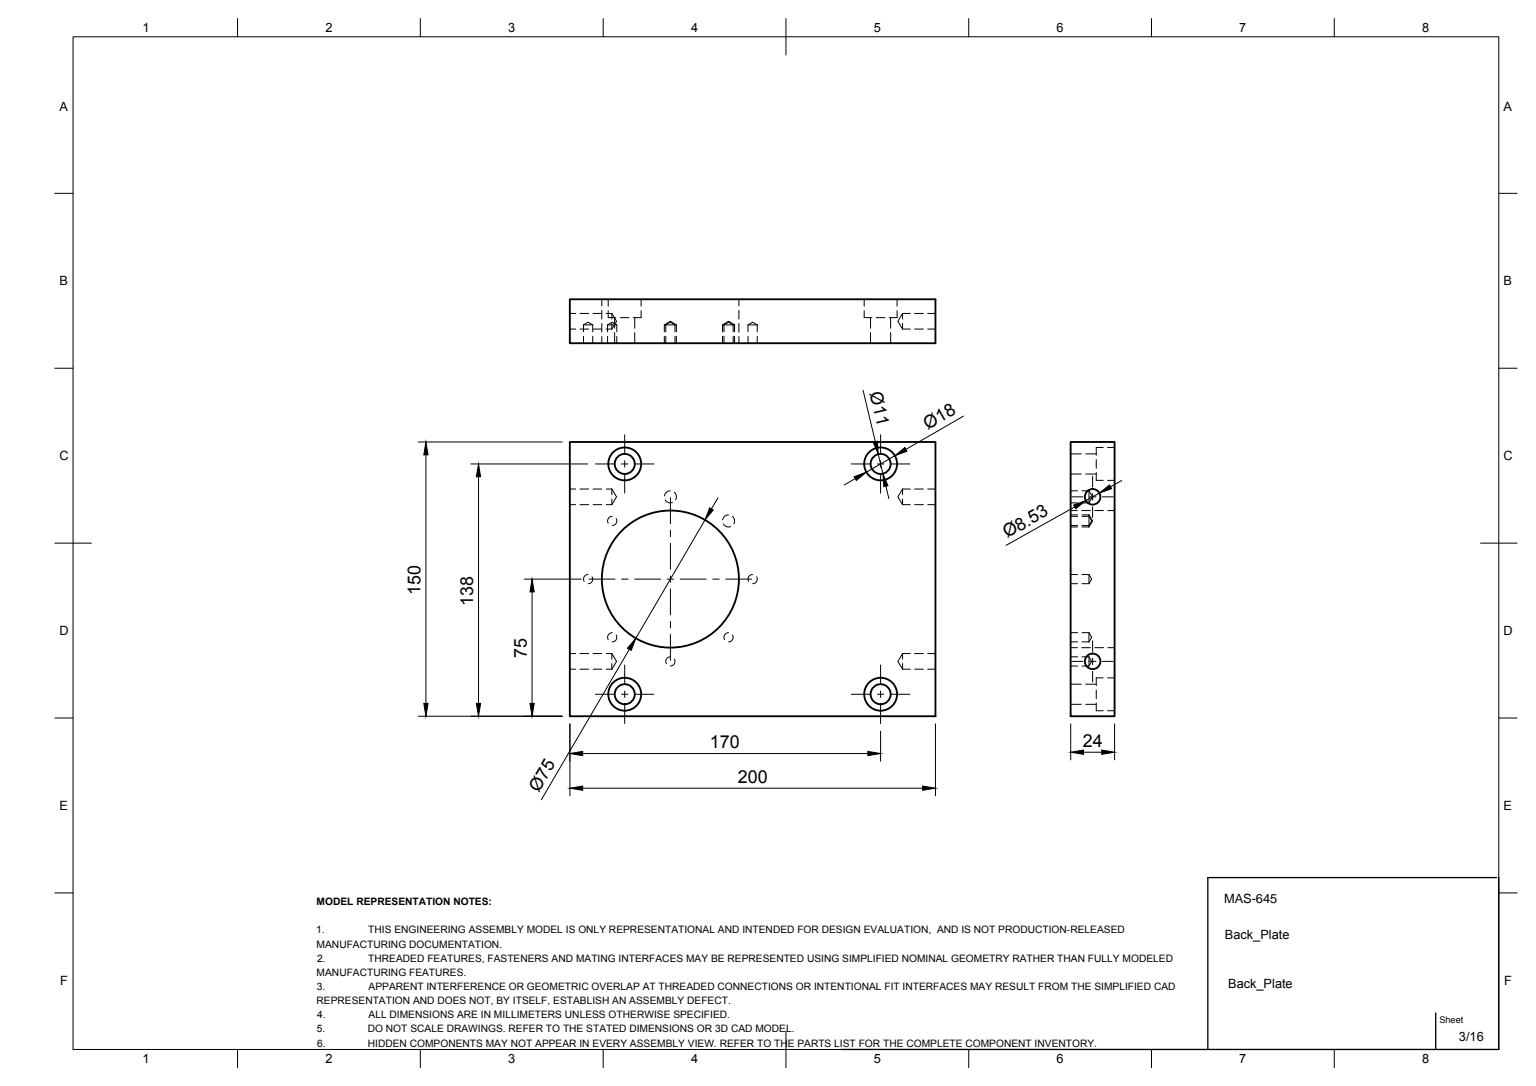
ISO-10303-21;
HEADER;
FILE_DESCRIPTION((''),'2;1');
FILE_NAME('Back_Plate.step','2026-10-09T10:54:55-07:00',(''),(''),'','','');
FILE_SCHEMA (('AUTOMOTIVE_DESIGN { 1 0 10303 214 3 1 1 }'));
ENDSEC;
DATA;
#10=MECHANICAL_DESIGN_GEOMETRIC_PRESENTATION_REPRESENTATION('',(#595),#63824);
#565=SHAPE_REPRESENTATION_RELATIONSHIP('SRR','None',#63879,#580) ;
#580=ADVANCED_BREP_SHAPE_REPRESENTATION('',(#610),#63809) ;
#595=STYLED_ITEM('',(#63963),#610) ;
#610=MANIFOLD_SOLID_BREP('Body1',#15494) ;
#625=FACE_BOUND('',#2415,.T.) ;
#626=FACE_BOUND('',#2419,.T.) ;
#627=FACE_BOUND('',#2423,.T.) ;
#628=FACE_BOUND('',#2427,.T.) ;
#629=FACE_BOUND('',#2448,.T.) ;
#630=FACE_BOUND('',#2449,.T.) ;
#631=FACE_BOUND('',#2452,.T.) ;
#632=FACE_BOUND('',#2453,.T.) ;
#633=FACE_BOUND('',#2456,.T.) ;
#634=FACE_BOUND('',#2457,.T.) ;
#635=FACE_BOUND('',#2458,.T.) ;
#636=FACE_BOUND('',#2459,.T.) ;
#637=FACE_BOUND('',#2460,.T.) ;
#638=FACE_BOUND('',#2462,.T.) ;
#639=FACE_BOUND('',#2463,.T.) ;
#640=FACE_BOUND('',#2464,.T.) ;
#641=FACE_BOUND('',#2465,.T.) ;
#642=FACE_BOUND('',#2466,.T.) ;
#643=FACE_BOUND('',#2467,.T.) ;
#644=FACE_BOUND('',#2468,.T.) ;
#645=FACE_BOUND('',#2469,.T.) ;
#646=FACE_BOUND('',#2470,.T.) ;
#647=FACE_BOUND('',#2471,.T.) ;
#648=FACE_BOUND('',#2472,.T.) ;
#649=FACE_BOUND('',#2473,.T.) ;
#650=FACE_BOUND('',#2474,.T.) ;
#832=PLANE('',#15693) ;
#833=PLANE('',#15700) ;
#834=PLANE('',#15707) ;
#835=PLANE('',#15714) ;
#836=PLANE('',#15756) ;
#837=PLANE('',#15757) ;
#838=PLANE('',#15758) ;
#839=PLANE('',#15759) ;
#840=PLANE('',#15760) ;
#841=PLANE('',#15761) ;
#1116=CYLINDRICAL_SURFACE('',#15679,4.263) ;
#1117=CYLINDRICAL_SURFACE('',#15683,4.263) ;
#1118=CYLINDRICAL_SURFACE('',#15687,4.263) ;
#1119=CYLINDRICAL_SURFACE('',#15691,4.263) ;
#1120=CYLINDRICAL_SURFACE('',#15696,9.) ;
#1121=CYLINDRICAL_SURFACE('',#15698,5.5) ;
#1122=CYLINDRICAL_SURFACE('',#15703,9.) ;
#1123=CYLINDRICAL_SURFACE('',#15705,5.5) ;
#1124=CYLINDRICAL_SURFACE('',#15710,9.) ;
#1125=CYLINDRICAL_SURFACE('',#15712,5.5) ;
#1126=CYLINDRICAL_SURFACE('',#15717,9.) ;
#1127=CYLINDRICAL_SURFACE('',#15719,5.5) ;
#1128=CYLINDRICAL_SURFACE('',#15723,3.3) ;
#1129=CYLINDRICAL_SURFACE('',#15727,2.5175) ;
#1130=CYLINDRICAL_SURFACE('',#15731,2.5175) ;
#1131=CYLINDRICAL_SURFACE('',#15735,2.5175) ;
#1132=CYLINDRICAL_SURFACE('',#15739,2.5175) ;
#1133=CYLINDRICAL_SURFACE('',#15743,2.5175) ;
#1134=CYLINDRICAL_SURFACE('',#15747,2.5175) ;
#1135=CYLINDRICAL_SURFACE('',#15751,3.3) ;
#1136=CYLINDRICAL_SURFACE('',#15753,37.5) ;
#1545=FACE_OUTER_BOUND('',#2406,.T.) ;
#1546=FACE_OUTER_BOUND('',#2407,.T.) ;
#1547=FACE_OUTER_BOUND('',#2408,.T.) ;
#1548=FACE_OUTER_BOUND('',#2409,.T.) ;
#1549=FACE_OUTER_BOUND('',#2410,.T.) ;
#1550=FACE_OUTER_BOUND('',#2411,.T.) ;
#1551=FACE_OUTER_BOUND('',#2412,.T.) ;
#1552=FACE_OUTER_BOUND('',#2413,.T.) ;
#1553=FACE_OUTER_BOUND('',#2414,.T.) ;
#1554=FACE_OUTER_BOUND('',#2416,.T.) ;
#1555=FACE_OUTER_BOUND('',#2417,.T.) ;
#1556=FACE_OUTER_BOUND('',#2418,.T.) ;
#1557=FACE_OUTER_BOUND('',#2420,.T.) ;
#1558=FACE_OUTER_BOUND('',#2421,.T.) ;
#1559=FACE_OUTER_BOUND('',#2422,.T.) ;
#1560=FACE_OUTER_BOUND('',#2424,.T.) ;
#1561=FACE_OUTER_BOUND('',#2425,.T.) ;
#1562=FACE_OUTER_BOUND('',#2426,.T.) ;
#1563=FACE_OUTER_BOUND('',#2428,.T.) ;
#1564=FACE_OUTER_BOUND('',#2429,.T.) ;
#1565=FACE_OUTER_BOUND('',#2430,.T.) ;
#1566=FACE_OUTER_BOUND('',#2431,.T.) ;
#1567=FACE_OUTER_BOUND('',#2432,.T.) ;
#1568=FACE_OUTER_BOUND('',#2433,.T.) ;
#1569=FACE_OUTER_BOUND('',#2434,.T.) ;
#1570=FACE_OUTER_BOUND('',#2435,.T.) ;
#1571=FACE_OUTER_BOUND('',#2436,.T.) ;
#1572=FACE_OUTER_BOUND('',#2437,.T.) ;
#1573=FACE_OUTER_BOUND('',#2438,.T.) ;
#1574=FACE_OUTER_BOUND('',#2439,.T.) ;
#1575=FACE_OUTER_BOUND('',#2440,.T.) ;
#1576=FACE_OUTER_BOUND('',#2441,.T.) ;
#1577=FACE_OUTER_BOUND('',#2442,.T.) ;
#1578=FACE_OUTER_BOUND('',#2443,.T.) ;
#1579=FACE_OUTER_BOUND('',#2444,.T.) ;
#1580=FACE_OUTER_BOUND('',#2445,.T.) ;
#1581=FACE_OUTER_BOUND('',#2446,.T.) ;
#1582=FACE_OUTER_BOUND('',#2447,.T.) ;
#1583=FACE_OUTER_BOUND('',#2450,.T.) ;
#1584=FACE_OUTER_BOUND('',#2451,.T.) ;
#1585=FACE_OUTER_BOUND('',#2454,.T.) ;
#1586=FACE_OUTER_BOUND('',#2455,.T.) ;
#1587=FACE_OUTER_BOUND('',#2461,.T.) ;
#2406=EDGE_LOOP('',(#9802,#9803,#9804)) ;
#2407=EDGE_LOOP('',(#9805,#9806,#9807,#9808)) ;
#2408=EDGE_LOOP('',(#9809,#9810,#9811)) ;
#2409=EDGE_LOOP('',(#9812,#9813,#9814,#9815)) ;
#2410=EDGE_LOOP('',(#9816,#9817,#9818)) ;
#2411=EDGE_LOOP('',(#9819,#9820,#9821,#9822)) ;
#2412=EDGE_LOOP('',(#9823,#9824,#9825)) ;
#2413=EDGE_LOOP('',(#9826,#9827,#9828,#9829)) ;
#2414=EDGE_LOOP('',(#9830)) ;
#2415=EDGE_LOOP('',(#9831)) ;
#2416=EDGE_LOOP('',(#9832,#9833,#9834,#9835)) ;
#2417=EDGE_LOOP('',(#9836,#9837,#9838,#9839)) ;
#2418=EDGE_LOOP('',(#9840)) ;
#2419=EDGE_LOOP('',(#9841)) ;
#2420=EDGE_LOOP('',(#9842,#9843,#9844,#9845)) ;
#2421=EDGE_LOOP('',(#9846,#9847,#9848,#9849)) ;
#2422=EDGE_LOOP('',(#9850)) ;
#2423=EDGE_LOOP('',(#9851)) ;
#2424=EDGE_LOOP('',(#9852,#9853,#9854,#9855)) ;
#2425=EDGE_LOOP('',(#9856,#9857,#9858,#9859)) ;
#2426=EDGE_LOOP('',(#9860)) ;
#2427=EDGE_LOOP('',(#9861)) ;
#2428=EDGE_LOOP('',(#9862,#9863,#9864,#9865)) ;
#2429=EDGE_LOOP('',(#9866,#9867,#9868,#9869)) ;
#2430=EDGE_LOOP('',(#9870,#9871,#9872)) ;
#2431=EDGE_LOOP('',(#9873,#9874,#9875,#9876)) ;
#2432=EDGE_LOOP('',(#9877,#9878,#9879)) ;
#2433=EDGE_LOOP('',(#9880,#9881,#9882,#9883)) ;
#2434=EDGE_LOOP('',(#9884,#9885,#9886)) ;
#2435=EDGE_LOOP('',(#9887,#9888,#9889,#9890)) ;
#2436=EDGE_LOOP('',(#9891,#9892,#9893)) ;
#2437=EDGE_LOOP('',(#9894,#9895,#9896,#9897)) ;
#2438=EDGE_LOOP('',(#9898,#9899,#9900)) ;
#2439=EDGE_LOOP('',(#9901,#9902,#9903,#9904)) ;
#2440=EDGE_LOOP('',(#9905,#9906,#9907)) ;
#2441=EDGE_LOOP('',(#9908,#9909,#9910,#9911)) ;
#2442=EDGE_LOOP('',(#9912,#9913,#9914)) ;
#2443=EDGE_LOOP('',(#9915,#9916,#9917,#9918)) ;
#2444=EDGE_LOOP('',(#9919,#9920,#9921)) ;
#2445=EDGE_LOOP('',(#9922,#9923,#9924,#9925)) ;
#2446=EDGE_LOOP('',(#9926,#9927,#9928,#9929)) ;
#2447=EDGE_LOOP('',(#9930,#9931,#9932,#9933)) ;
#2448=EDGE_LOOP('',(#9934)) ;
#2449=EDGE_LOOP('',(#9935)) ;
#2450=EDGE_LOOP('',(#9936,#9937,#9938,#9939)) ;
#2451=EDGE_LOOP('',(#9940,#9941,#9942,#9943)) ;
#2452=EDGE_LOOP('',(#9944)) ;
#2453=EDGE_LOOP('',(#9945)) ;
#2454=EDGE_LOOP('',(#9946,#9947,#9948,#9949)) ;
#2455=EDGE_LOOP('',(#9950,#9951,#9952,#9953)) ;
#2456=EDGE_LOOP('',(#9954)) ;
#2457=EDGE_LOOP('',(#9955)) ;
#2458=EDGE_LOOP('',(#9956)) ;
#2459=EDGE_LOOP('',(#9957)) ;
#2460=EDGE_LOOP('',(#9958)) ;
#2461=EDGE_LOOP('',(#9959,#9960,#9961,#9962)) ;
#2462=EDGE_LOOP('',(#9963)) ;
#2463=EDGE_LOOP('',(#9964)) ;
#2464=EDGE_LOOP('',(#9965)) ;
#2465=EDGE_LOOP('',(#9966)) ;
#2466=EDGE_LOOP('',(#9967)) ;
#2467=EDGE_LOOP('',(#9968)) ;
#2468=EDGE_LOOP('',(#9969)) ;
#2469=EDGE_LOOP('',(#9970)) ;
#2470=EDGE_LOOP('',(#9971)) ;
#2471=EDGE_LOOP('',(#9972)) ;
#2472=EDGE_LOOP('',(#9973)) ;
#2473=EDGE_LOOP('',(#9974)) ;
#2474=EDGE_LOOP('',(#9975)) ;
#3474=CIRCLE('',#15678,4.263) ;
#3475=CIRCLE('',#15680,4.263) ;
#3476=CIRCLE('',#15682,4.263) ;
#3477=CIRCLE('',#15684,4.263) ;
#3478=CIRCLE('',#15686,4.263) ;
#3479=CIRCLE('',#15688,4.263) ;
#3480=CIRCLE('',#15690,4.263) ;
#3481=CIRCLE('',#15692,4.263) ;
#3482=CIRCLE('',#15694,9.) ;
#3483=CIRCLE('',#15695,5.5) ;
#3484=CIRCLE('',#15697,9.) ;
#3485=CIRCLE('',#15699,5.5) ;
#3486=CIRCLE('',#15701,9.) ;
#3487=CIRCLE('',#15702,5.5) ;
#3488=CIRCLE('',#15704,9.) ;
#3489=CIRCLE('',#15706,5.5) ;
#3490=CIRCLE('',#15708,9.) ;
#3491=CIRCLE('',#15709,5.5) ;
#3492=CIRCLE('',#15711,9.) ;
#3493=CIRCLE('',#15713,5.5) ;
#3494=CIRCLE('',#15715,9.) ;
#3495=CIRCLE('',#15716,5.5) ;
#3496=CIRCLE('',#15718,9.) ;
#3497=CIRCLE('',#15720,5.5) ;
#3498=CIRCLE('',#15722,3.3) ;
#3499=CIRCLE('',#15724,3.3) ;
#3500=CIRCLE('',#15726,2.5175) ;
#3501=CIRCLE('',#15728,2.5175) ;
#3502=CIRCLE('',#15730,2.5175) ;
#3503=CIRCLE('',#15732,2.5175) ;
#3504=CIRCLE('',#15734,2.5175) ;
#3505=CIRCLE('',#15736,2.5175) ;
#3506=CIRCLE('',#15738,2.5175) ;
#3507=CIRCLE('',#15740,2.5175) ;
#3508=CIRCLE('',#15742,2.5175) ;
#3509=CIRCLE('',#15744,2.5175) ;
#3510=CIRCLE('',#15746,2.5175) ;
#3511=CIRCLE('',#15748,2.5175) ;
#3512=CIRCLE('',#15750,3.3) ;
#3513=CIRCLE('',#15752,3.3) ;
#3514=CIRCLE('',#15754,37.5) ;
#3515=CIRCLE('',#15755,37.5) ;
#4690=LINE('',#23017,#5346) ;
#4691=LINE('',#23022,#5347) ;
#4692=LINE('',#23026,#5348) ;
#4693=LINE('',#23031,#5349) ;
#4694=LINE('',#23035,#5350) ;
#4695=LINE('',#23040,#5351) ;
#4696=LINE('',#23044,#5352) ;
#4697=LINE('',#23049,#5353) ;
#4698=LINE('',#23058,#5354) ;
#4699=LINE('',#23061,#5355) ;
#4700=LINE('',#23071,#5356) ;
#4701=LINE('',#23074,#5357) ;
#4702=LINE('',#23084,#5358) ;
#4703=LINE('',#23087,#5359) ;
#4704=LINE('',#23097,#5360) ;
#4705=LINE('',#23100,#5361) ;
#4706=LINE('',#23105,#5362) ;
#4707=LINE('',#23110,#5363) ;
#4708=LINE('',#23114,#5364) ;
#4709=LINE('',#23119,#5365) ;
#4710=LINE('',#23123,#5366) ;
#4711=LINE('',#23128,#5367) ;
#4712=LINE('',#23132,#5368) ;
#4713=LINE('',#23137,#5369) ;
#4714=LINE('',#23141,#5370) ;
#4715=LINE('',#23146,#5371) ;
#4716=LINE('',#23150,#5372) ;
#4717=LINE('',#23155,#5373) ;
#4718=LINE('',#23159,#5374) ;
#4719=LINE('',#23164,#5375) ;
#4720=LINE('',#23168,#5376) ;
#4721=LINE('',#23173,#5377) ;
#4722=LINE('',#23178,#5378) ;
#4723=LINE('',#23183,#5379) ;
#4724=LINE('',#23185,#5380) ;
#4725=LINE('',#23187,#5381) ;
#4726=LINE('',#23188,#5382) ;
#4727=LINE('',#23191,#5383) ;
#4728=LINE('',#23193,#5384) ;
#4729=LINE('',#23194,#5385) ;
#4730=LINE('',#23197,#5386) ;
#4731=LINE('',#23199,#5387) ;
#4732=LINE('',#23200,#5388) ;
#4733=LINE('',#23202,#5389) ;
#4734=LINE('',#23203,#5390) ;
#5346=VECTOR('',#17908,2.42186816158307) ;
#5347=VECTOR('',#17915,4.263) ;
#5348=VECTOR('',#17918,2.42186816158307) ;
#5349=VECTOR('',#17925,4.263) ;
#5350=VECTOR('',#17928,2.42186816158307) ;
#5351=VECTOR('',#17935,4.263) ;
#5352=VECTOR('',#17938,2.42186816158307) ;
#5353=VECTOR('',#17945,4.263) ;
#5354=VECTOR('',#17956,9.) ;
#5355=VECTOR('',#17959,5.5) ;
#5356=VECTOR('',#17972,9.) ;
#5357=VECTOR('',#17975,5.5) ;
#5358=VECTOR('',#17988,9.) ;
#5359=VECTOR('',#17991,5.5) ;
#5360=VECTOR('',#18004,9.) ;
#5361=VECTOR('',#18007,5.5) ;
#5362=VECTOR('',#18012,1.65) ;
#5363=VECTOR('',#18019,3.3) ;
#5364=VECTOR('',#18022,1.44243074893998) ;
#5365=VECTOR('',#18029,2.5175) ;
#5366=VECTOR('',#18032,1.44243074893998) ;
#5367=VECTOR('',#18039,2.5175) ;
#5368=VECTOR('',#18042,1.44243074893998) ;
#5369=VECTOR('',#18049,2.5175) ;
#5370=VECTOR('',#18052,1.44243074893998) ;
#5371=VECTOR('',#18059,2.5175) ;
#5372=VECTOR('',#18062,1.44243074893998) ;
#5373=VECTOR('',#18069,2.5175) ;
#5374=VECTOR('',#18072,1.44243074893998) ;
#5375=VECTOR('',#18079,2.5175) ;
#5376=VECTOR('',#18082,1.65) ;
#5377=VECTOR('',#18089,3.3) ;
#5378=VECTOR('',#18094,37.5) ;
#5379=VECTOR('',#18099,10.) ;
#5380=VECTOR('',#18100,10.) ;
#5381=VECTOR('',#18101,10.) ;
#5382=VECTOR('',#18102,10.) ;
#5383=VECTOR('',#18105,10.) ;
#5384=VECTOR('',#18106,10.) ;
#5385=VECTOR('',#18107,10.) ;
#5386=VECTOR('',#18110,10.) ;
#5387=VECTOR('',#18111,10.) ;
#5388=VECTOR('',#18112,10.) ;
#5389=VECTOR('',#18115,10.) ;
#5390=VECTOR('',#18116,10.) ;
#6002=VERTEX_POINT('',#23015) ;
#6003=VERTEX_POINT('',#23016) ;
#6004=VERTEX_POINT('',#23020) ;
#6005=VERTEX_POINT('',#23024) ;
#6006=VERTEX_POINT('',#23025) ;
#6007=VERTEX_POINT('',#23029) ;
#6008=VERTEX_POINT('',#23033) ;
#6009=VERTEX_POINT('',#23034) ;
#6010=VERTEX_POINT('',#23038) ;
#6011=VERTEX_POINT('',#23042) ;
#6012=VERTEX_POINT('',#23043) ;
#6013=VERTEX_POINT('',#23047) ;
#6014=VERTEX_POINT('',#23051) ;
#6015=VERTEX_POINT('',#23053) ;
#6016=VERTEX_POINT('',#23056) ;
#6017=VERTEX_POINT('',#23060) ;
#6018=VERTEX_POINT('',#23064) ;
#6019=VERTEX_POINT('',#23066) ;
#6020=VERTEX_POINT('',#23069) ;
#6021=VERTEX_POINT('',#23073) ;
#6022=VERTEX_POINT('',#23077) ;
#6023=VERTEX_POINT('',#23079) ;
#6024=VERTEX_POINT('',#23082) ;
#6025=VERTEX_POINT('',#23086) ;
#6026=VERTEX_POINT('',#23090) ;
#6027=VERTEX_POINT('',#23092) ;
#6028=VERTEX_POINT('',#23095) ;
#6029=VERTEX_POINT('',#23099) ;
#6030=VERTEX_POINT('',#23103) ;
#6031=VERTEX_POINT('',#23104) ;
#6032=VERTEX_POINT('',#23108) ;
#6033=VERTEX_POINT('',#23112) ;
#6034=VERTEX_POINT('',#23113) ;
#6035=VERTEX_POINT('',#23117) ;
#6036=VERTEX_POINT('',#23121) ;
#6037=VERTEX_POINT('',#23122) ;
#6038=VERTEX_POINT('',#23126) ;
#6039=VERTEX_POINT('',#23130) ;
#6040=VERTEX_POINT('',#23131) ;
#6041=VERTEX_POINT('',#23135) ;
#6042=VERTEX_POINT('',#23139) ;
#6043=VERTEX_POINT('',#23140) ;
#6044=VERTEX_POINT('',#23144) ;
#6045=VERTEX_POINT('',#23148) ;
#6046=VERTEX_POINT('',#23149) ;
#6047=VERTEX_POINT('',#23153) ;
#6048=VERTEX_POINT('',#23157) ;
#6049=VERTEX_POINT('',#23158) ;
#6050=VERTEX_POINT('',#23162) ;
#6051=VERTEX_POINT('',#23166) ;
#6052=VERTEX_POINT('',#23167) ;
#6053=VERTEX_POINT('',#23171) ;
#6054=VERTEX_POINT('',#23175) ;
#6055=VERTEX_POINT('',#23177) ;
#6056=VERTEX_POINT('',#23181) ;
#6057=VERTEX_POINT('',#23182) ;
#6058=VERTEX_POINT('',#23184) ;
#6059=VERTEX_POINT('',#23186) ;
#6060=VERTEX_POINT('',#23190) ;
#6061=VERTEX_POINT('',#23192) ;
#6062=VERTEX_POINT('',#23196) ;
#6063=VERTEX_POINT('',#23198) ;
#7455=EDGE_CURVE('',#6002,#6003,#4690,.T.) ;
#7456=EDGE_CURVE('',#6003,#6003,#3474,.T.) ;
#7457=EDGE_CURVE('',#6004,#6004,#3475,.T.) ;
#7458=EDGE_CURVE('',#6004,#6003,#4691,.T.) ;
#7459=EDGE_CURVE('',#6005,#6006,#4692,.T.) ;
#7460=EDGE_CURVE('',#6006,#6006,#3476,.T.) ;
#7461=EDGE_CURVE('',#6007,#6007,#3477,.T.) ;
#7462=EDGE_CURVE('',#6007,#6006,#4693,.T.) ;
#7463=EDGE_CURVE('',#6008,#6009,#4694,.T.) ;
#7464=EDGE_CURVE('',#6009,#6009,#3478,.T.) ;
#7465=EDGE_CURVE('',#6010,#6010,#3479,.T.) ;
#7466=EDGE_CURVE('',#6010,#6009,#4695,.T.) ;
#7467=EDGE_CURVE('',#6011,#6012,#4696,.T.) ;
#7468=EDGE_CURVE('',#6012,#6012,#3480,.T.) ;
#7469=EDGE_CURVE('',#6013,#6013,#3481,.T.) ;
#7470=EDGE_CURVE('',#6013,#6012,#4697,.T.) ;
#7471=EDGE_CURVE('',#6014,#6014,#3482,.T.) ;
#7472=EDGE_CURVE('',#6015,#6015,#3483,.T.) ;
#7473=EDGE_CURVE('',#6016,#6016,#3484,.T.) ;
#7474=EDGE_CURVE('',#6016,#6014,#4698,.T.) ;
#7475=EDGE_CURVE('',#6015,#6017,#4699,.T.) ;
#7476=EDGE_CURVE('',#6017,#6017,#3485,.T.) ;
#7477=EDGE_CURVE('',#6018,#6018,#3486,.T.) ;
#7478=EDGE_CURVE('',#6019,#6019,#3487,.T.) ;
#7479=EDGE_CURVE('',#6020,#6020,#3488,.T.) ;
#7480=EDGE_CURVE('',#6020,#6018,#4700,.T.) ;
#7481=EDGE_CURVE('',#6019,#6021,#4701,.T.) ;
#7482=EDGE_CURVE('',#6021,#6021,#3489,.T.) ;
#7483=EDGE_CURVE('',#6022,#6022,#3490,.T.) ;
#7484=EDGE_CURVE('',#6023,#6023,#3491,.T.) ;
#7485=EDGE_CURVE('',#6024,#6024,#3492,.T.) ;
#7486=EDGE_CURVE('',#6024,#6022,#4702,.T.) ;
#7487=EDGE_CURVE('',#6023,#6025,#4703,.T.) ;
#7488=EDGE_CURVE('',#6025,#6025,#3493,.T.) ;
#7489=EDGE_CURVE('',#6026,#6026,#3494,.T.) ;
#7490=EDGE_CURVE('',#6027,#6027,#3495,.T.) ;
#7491=EDGE_CURVE('',#6028,#6028,#3496,.T.) ;
#7492=EDGE_CURVE('',#6028,#6026,#4704,.T.) ;
#7493=EDGE_CURVE('',#6027,#6029,#4705,.T.) ;
#7494=EDGE_CURVE('',#6029,#6029,#3497,.T.) ;
#7495=EDGE_CURVE('',#6030,#6031,#4706,.T.) ;
#7496=EDGE_CURVE('',#6031,#6031,#3498,.T.) ;
#7497=EDGE_CURVE('',#6032,#6032,#3499,.T.) ;
#7498=EDGE_CURVE('',#6032,#6031,#4707,.T.) ;
#7499=EDGE_CURVE('',#6033,#6034,#4708,.T.) ;
#7500=EDGE_CURVE('',#6034,#6034,#3500,.T.) ;
#7501=EDGE_CURVE('',#6035,#6035,#3501,.F.) ;
#7502=EDGE_CURVE('',#6035,#6034,#4709,.T.) ;
#7503=EDGE_CURVE('',#6036,#6037,#4710,.T.) ;
#7504=EDGE_CURVE('',#6037,#6037,#3502,.T.) ;
#7505=EDGE_CURVE('',#6038,#6038,#3503,.F.) ;
#7506=EDGE_CURVE('',#6038,#6037,#4711,.T.) ;
#7507=EDGE_CURVE('',#6039,#6040,#4712,.T.) ;
#7508=EDGE_CURVE('',#6040,#6040,#3504,.T.) ;
#7509=EDGE_CURVE('',#6041,#6041,#3505,.F.) ;
#7510=EDGE_CURVE('',#6041,#6040,#4713,.T.) ;
#7511=EDGE_CURVE('',#6042,#6043,#4714,.T.) ;
#7512=EDGE_CURVE('',#6043,#6043,#3506,.T.) ;
#7513=EDGE_CURVE('',#6044,#6044,#3507,.F.) ;
#7514=EDGE_CURVE('',#6044,#6043,#4715,.T.) ;
#7515=EDGE_CURVE('',#6045,#6046,#4716,.T.) ;
#7516=EDGE_CURVE('',#6046,#6046,#3508,.T.) ;
#7517=EDGE_CURVE('',#6047,#6047,#3509,.F.) ;
#7518=EDGE_CURVE('',#6047,#6046,#4717,.T.) ;
#7519=EDGE_CURVE('',#6048,#6049,#4718,.T.) ;
#7520=EDGE_CURVE('',#6049,#6049,#3510,.T.) ;
#7521=EDGE_CURVE('',#6050,#6050,#3511,.F.) ;
#7522=EDGE_CURVE('',#6050,#6049,#4719,.T.) ;
#7523=EDGE_CURVE('',#6051,#6052,#4720,.T.) ;
#7524=EDGE_CURVE('',#6052,#6052,#3512,.T.) ;
#7525=EDGE_CURVE('',#6053,#6053,#3513,.T.) ;
#7526=EDGE_CURVE('',#6053,#6052,#4721,.T.) ;
#7527=EDGE_CURVE('',#6054,#6054,#3514,.T.) ;
#7528=EDGE_CURVE('',#6054,#6055,#4722,.T.) ;
#7529=EDGE_CURVE('',#6055,#6055,#3515,.T.) ;
#7530=EDGE_CURVE('',#6056,#6057,#4723,.T.) ;
#7531=EDGE_CURVE('',#6056,#6058,#4724,.T.) ;
#7532=EDGE_CURVE('',#6059,#6058,#4725,.T.) ;
#7533=EDGE_CURVE('',#6057,#6059,#4726,.T.) ;
#7534=EDGE_CURVE('',#6057,#6060,#4727,.T.) ;
#7535=EDGE_CURVE('',#6061,#6059,#4728,.T.) ;
#7536=EDGE_CURVE('',#6060,#6061,#4729,.T.) ;
#7537=EDGE_CURVE('',#6062,#6060,#4730,.T.) ;
#7538=EDGE_CURVE('',#6063,#6061,#4731,.T.) ;
#7539=EDGE_CURVE('',#6062,#6063,#4732,.T.) ;
#7540=EDGE_CURVE('',#6062,#6056,#4733,.T.) ;
#7541=EDGE_CURVE('',#6058,#6063,#4734,.T.) ;
#9802=ORIENTED_EDGE('',*,*,#7455,.T.) ;
#9803=ORIENTED_EDGE('',*,*,#7456,.F.) ;
#9804=ORIENTED_EDGE('',*,*,#7455,.F.) ;
#9805=ORIENTED_EDGE('',*,*,#7457,.F.) ;
#9806=ORIENTED_EDGE('',*,*,#7458,.T.) ;
#9807=ORIENTED_EDGE('',*,*,#7456,.T.) ;
#9808=ORIENTED_EDGE('',*,*,#7458,.F.) ;
#9809=ORIENTED_EDGE('',*,*,#7459,.T.) ;
#9810=ORIENTED_EDGE('',*,*,#7460,.F.) ;
#9811=ORIENTED_EDGE('',*,*,#7459,.F.) ;
#9812=ORIENTED_EDGE('',*,*,#7461,.F.) ;
#9813=ORIENTED_EDGE('',*,*,#7462,.T.) ;
#9814=ORIENTED_EDGE('',*,*,#7460,.T.) ;
#9815=ORIENTED_EDGE('',*,*,#7462,.F.) ;
#9816=ORIENTED_EDGE('',*,*,#7463,.T.) ;
#9817=ORIENTED_EDGE('',*,*,#7464,.F.) ;
#9818=ORIENTED_EDGE('',*,*,#7463,.F.) ;
#9819=ORIENTED_EDGE('',*,*,#7465,.F.) ;
#9820=ORIENTED_EDGE('',*,*,#7466,.T.) ;
#9821=ORIENTED_EDGE('',*,*,#7464,.T.) ;
#9822=ORIENTED_EDGE('',*,*,#7466,.F.) ;
#9823=ORIENTED_EDGE('',*,*,#7467,.T.) ;
#9824=ORIENTED_EDGE('',*,*,#7468,.F.) ;
#9825=ORIENTED_EDGE('',*,*,#7467,.F.) ;
#9826=ORIENTED_EDGE('',*,*,#7469,.F.) ;
#9827=ORIENTED_EDGE('',*,*,#7470,.T.) ;
#9828=ORIENTED_EDGE('',*,*,#7468,.T.) ;
#9829=ORIENTED_EDGE('',*,*,#7470,.F.) ;
#9830=ORIENTED_EDGE('',*,*,#7471,.F.) ;
#9831=ORIENTED_EDGE('',*,*,#7472,.T.) ;
#9832=ORIENTED_EDGE('',*,*,#7473,.F.) ;
#9833=ORIENTED_EDGE('',*,*,#7474,.T.) ;
#9834=ORIENTED_EDGE('',*,*,#7471,.T.) ;
#9835=ORIENTED_EDGE('',*,*,#7474,.F.) ;
#9836=ORIENTED_EDGE('',*,*,#7472,.F.) ;
#9837=ORIENTED_EDGE('',*,*,#7475,.T.) ;
#9838=ORIENTED_EDGE('',*,*,#7476,.F.) ;
#9839=ORIENTED_EDGE('',*,*,#7475,.F.) ;
#9840=ORIENTED_EDGE('',*,*,#7477,.F.) ;
#9841=ORIENTED_EDGE('',*,*,#7478,.T.) ;
#9842=ORIENTED_EDGE('',*,*,#7479,.F.) ;
#9843=ORIENTED_EDGE('',*,*,#7480,.T.) ;
#9844=ORIENTED_EDGE('',*,*,#7477,.T.) ;
#9845=ORIENTED_EDGE('',*,*,#7480,.F.) ;
#9846=ORIENTED_EDGE('',*,*,#7478,.F.) ;
#9847=ORIENTED_EDGE('',*,*,#7481,.T.) ;
#9848=ORIENTED_EDGE('',*,*,#7482,.F.) ;
#9849=ORIENTED_EDGE('',*,*,#7481,.F.) ;
#9850=ORIENTED_EDGE('',*,*,#7483,.F.) ;
#9851=ORIENTED_EDGE('',*,*,#7484,.T.) ;
#9852=ORIENTED_EDGE('',*,*,#7485,.F.) ;
#9853=ORIENTED_EDGE('',*,*,#7486,.T.) ;
#9854=ORIENTED_EDGE('',*,*,#7483,.T.) ;
#9855=ORIENTED_EDGE('',*,*,#7486,.F.) ;
#9856=ORIENTED_EDGE('',*,*,#7484,.F.) ;
#9857=ORIENTED_EDGE('',*,*,#7487,.T.) ;
#9858=ORIENTED_EDGE('',*,*,#7488,.F.) ;
#9859=ORIENTED_EDGE('',*,*,#7487,.F.) ;
#9860=ORIENTED_EDGE('',*,*,#7489,.F.) ;
#9861=ORIENTED_EDGE('',*,*,#7490,.T.) ;
#9862=ORIENTED_EDGE('',*,*,#7491,.F.) ;
#9863=ORIENTED_EDGE('',*,*,#7492,.T.) ;
#9864=ORIENTED_EDGE('',*,*,#7489,.T.) ;
#9865=ORIENTED_EDGE('',*,*,#7492,.F.) ;
#9866=ORIENTED_EDGE('',*,*,#7490,.F.) ;
#9867=ORIENTED_EDGE('',*,*,#7493,.T.) ;
#9868=ORIENTED_EDGE('',*,*,#7494,.F.) ;
#9869=ORIENTED_EDGE('',*,*,#7493,.F.) ;
#9870=ORIENTED_EDGE('',*,*,#7495,.T.) ;
#9871=ORIENTED_EDGE('',*,*,#7496,.F.) ;
#9872=ORIENTED_EDGE('',*,*,#7495,.F.) ;
#9873=ORIENTED_EDGE('',*,*,#7497,.F.) ;
#9874=ORIENTED_EDGE('',*,*,#7498,.T.) ;
#9875=ORIENTED_EDGE('',*,*,#7496,.T.) ;
#9876=ORIENTED_EDGE('',*,*,#7498,.F.) ;
#9877=ORIENTED_EDGE('',*,*,#7499,.T.) ;
#9878=ORIENTED_EDGE('',*,*,#7500,.F.) ;
#9879=ORIENTED_EDGE('',*,*,#7499,.F.) ;
#9880=ORIENTED_EDGE('',*,*,#7501,.F.) ;
#9881=ORIENTED_EDGE('',*,*,#7502,.T.) ;
#9882=ORIENTED_EDGE('',*,*,#7500,.T.) ;
#9883=ORIENTED_EDGE('',*,*,#7502,.F.) ;
#9884=ORIENTED_EDGE('',*,*,#7503,.T.) ;
#9885=ORIENTED_EDGE('',*,*,#7504,.F.) ;
#9886=ORIENTED_EDGE('',*,*,#7503,.F.) ;
#9887=ORIENTED_EDGE('',*,*,#7505,.F.) ;
#9888=ORIENTED_EDGE('',*,*,#7506,.T.) ;
#9889=ORIENTED_EDGE('',*,*,#7504,.T.) ;
#9890=ORIENTED_EDGE('',*,*,#7506,.F.) ;
#9891=ORIENTED_EDGE('',*,*,#7507,.T.) ;
#9892=ORIENTED_EDGE('',*,*,#7508,.F.) ;
#9893=ORIENTED_EDGE('',*,*,#7507,.F.) ;
#9894=ORIENTED_EDGE('',*,*,#7509,.F.) ;
#9895=ORIENTED_EDGE('',*,*,#7510,.T.) ;
#9896=ORIENTED_EDGE('',*,*,#7508,.T.) ;
#9897=ORIENTED_EDGE('',*,*,#7510,.F.) ;
#9898=ORIENTED_EDGE('',*,*,#7511,.T.) ;
#9899=ORIENTED_EDGE('',*,*,#7512,.F.) ;
#9900=ORIENTED_EDGE('',*,*,#7511,.F.) ;
#9901=ORIENTED_EDGE('',*,*,#7513,.F.) ;
#9902=ORIENTED_EDGE('',*,*,#7514,.T.) ;
#9903=ORIENTED_EDGE('',*,*,#7512,.T.) ;
#9904=ORIENTED_EDGE('',*,*,#7514,.F.) ;
#9905=ORIENTED_EDGE('',*,*,#7515,.T.) ;
#9906=ORIENTED_EDGE('',*,*,#7516,.F.) ;
#9907=ORIENTED_EDGE('',*,*,#7515,.F.) ;
#9908=ORIENTED_EDGE('',*,*,#7517,.F.) ;
#9909=ORIENTED_EDGE('',*,*,#7518,.T.) ;
#9910=ORIENTED_EDGE('',*,*,#7516,.T.) ;
#9911=ORIENTED_EDGE('',*,*,#7518,.F.) ;
#9912=ORIENTED_EDGE('',*,*,#7519,.T.) ;
#9913=ORIENTED_EDGE('',*,*,#7520,.F.) ;
#9914=ORIENTED_EDGE('',*,*,#7519,.F.) ;
#9915=ORIENTED_EDGE('',*,*,#7521,.F.) ;
#9916=ORIENTED_EDGE('',*,*,#7522,.T.) ;
#9917=ORIENTED_EDGE('',*,*,#7520,.T.) ;
#9918=ORIENTED_EDGE('',*,*,#7522,.F.) ;
#9919=ORIENTED_EDGE('',*,*,#7523,.T.) ;
#9920=ORIENTED_EDGE('',*,*,#7524,.F.) ;
#9921=ORIENTED_EDGE('',*,*,#7523,.F.) ;
#9922=ORIENTED_EDGE('',*,*,#7525,.F.) ;
#9923=ORIENTED_EDGE('',*,*,#7526,.T.) ;
#9924=ORIENTED_EDGE('',*,*,#7524,.T.) ;
#9925=ORIENTED_EDGE('',*,*,#7526,.F.) ;
#9926=ORIENTED_EDGE('',*,*,#7527,.F.) ;
#9927=ORIENTED_EDGE('',*,*,#7528,.T.) ;
#9928=ORIENTED_EDGE('',*,*,#7529,.F.) ;
#9929=ORIENTED_EDGE('',*,*,#7528,.F.) ;
#9930=ORIENTED_EDGE('',*,*,#7530,.F.) ;
#9931=ORIENTED_EDGE('',*,*,#7531,.T.) ;
#9932=ORIENTED_EDGE('',*,*,#7532,.F.) ;
#9933=ORIENTED_EDGE('',*,*,#7533,.F.) ;
#9934=ORIENTED_EDGE('',*,*,#7465,.T.) ;
#9935=ORIENTED_EDGE('',*,*,#7469,.T.) ;
#9936=ORIENTED_EDGE('',*,*,#7534,.F.) ;
#9937=ORIENTED_EDGE('',*,*,#7533,.T.) ;
#9938=ORIENTED_EDGE('',*,*,#7535,.F.) ;
#9939=ORIENTED_EDGE('',*,*,#7536,.F.) ;
#9940=ORIENTED_EDGE('',*,*,#7537,.T.) ;
#9941=ORIENTED_EDGE('',*,*,#7536,.T.) ;
#9942=ORIENTED_EDGE('',*,*,#7538,.F.) ;
#9943=ORIENTED_EDGE('',*,*,#7539,.F.) ;
#9944=ORIENTED_EDGE('',*,*,#7457,.T.) ;
#9945=ORIENTED_EDGE('',*,*,#7461,.T.) ;
#9946=ORIENTED_EDGE('',*,*,#7540,.F.) ;
#9947=ORIENTED_EDGE('',*,*,#7539,.T.) ;
#9948=ORIENTED_EDGE('',*,*,#7541,.F.) ;
#9949=ORIENTED_EDGE('',*,*,#7531,.F.) ;
#9950=ORIENTED_EDGE('',*,*,#7540,.T.) ;
#9951=ORIENTED_EDGE('',*,*,#7530,.T.) ;
#9952=ORIENTED_EDGE('',*,*,#7534,.T.) ;
#9953=ORIENTED_EDGE('',*,*,#7537,.F.) ;
#9954=ORIENTED_EDGE('',*,*,#7473,.T.) ;
#9955=ORIENTED_EDGE('',*,*,#7479,.T.) ;
#9956=ORIENTED_EDGE('',*,*,#7485,.T.) ;
#9957=ORIENTED_EDGE('',*,*,#7491,.T.) ;
#9958=ORIENTED_EDGE('',*,*,#7527,.T.) ;
#9959=ORIENTED_EDGE('',*,*,#7541,.T.) ;
#9960=ORIENTED_EDGE('',*,*,#7538,.T.) ;
#9961=ORIENTED_EDGE('',*,*,#7535,.T.) ;
#9962=ORIENTED_EDGE('',*,*,#7532,.T.) ;
#9963=ORIENTED_EDGE('',*,*,#7476,.T.) ;
#9964=ORIENTED_EDGE('',*,*,#7482,.T.) ;
#9965=ORIENTED_EDGE('',*,*,#7488,.T.) ;
#9966=ORIENTED_EDGE('',*,*,#7494,.T.) ;
#9967=ORIENTED_EDGE('',*,*,#7497,.T.) ;
#9968=ORIENTED_EDGE('',*,*,#7501,.T.) ;
#9969=ORIENTED_EDGE('',*,*,#7505,.T.) ;
#9970=ORIENTED_EDGE('',*,*,#7509,.T.) ;
#9971=ORIENTED_EDGE('',*,*,#7513,.T.) ;
#9972=ORIENTED_EDGE('',*,*,#7517,.T.) ;
#9973=ORIENTED_EDGE('',*,*,#7521,.T.) ;
#9974=ORIENTED_EDGE('',*,*,#7525,.T.) ;
#9975=ORIENTED_EDGE('',*,*,#7529,.T.) ;
#14496=CONICAL_SURFACE('',#15677,2.42186816158307,1.02974425867665) ;
#14497=CONICAL_SURFACE('',#15681,2.42186816158307,1.02974425867665) ;
#14498=CONICAL_SURFACE('',#15685,2.42186816158307,1.02974425867665) ;
#14499=CONICAL_SURFACE('',#15689,2.42186816158307,1.02974425867665) ;
#14500=CONICAL_SURFACE('',#15721,1.65,1.02974425867665) ;
#14501=CONICAL_SURFACE('',#15725,1.44243074893998,1.02974425867665) ;
#14502=CONICAL_SURFACE('',#15729,1.44243074893998,1.02974425867665) ;
#14503=CONICAL_SURFACE('',#15733,1.44243074893998,1.02974425867665) ;
#14504=CONICAL_SURFACE('',#15737,1.44243074893998,1.02974425867665) ;
#14505=CONICAL_SURFACE('',#15741,1.44243074893998,1.02974425867665) ;
#14506=CONICAL_SURFACE('',#15745,1.44243074893998,1.02974425867665) ;
#14507=CONICAL_SURFACE('',#15749,1.65,1.02974425867665) ;
#14633=ADVANCED_FACE('',(#1545),#14496,.F.) ;
#14634=ADVANCED_FACE('',(#1546),#1116,.F.) ;
#14635=ADVANCED_FACE('',(#1547),#14497,.F.) ;
#14636=ADVANCED_FACE('',(#1548),#1117,.F.) ;
#14637=ADVANCED_FACE('',(#1549),#14498,.F.) ;
#14638=ADVANCED_FACE('',(#1550),#1118,.F.) ;
#14639=ADVANCED_FACE('',(#1551),#14499,.F.) ;
#14640=ADVANCED_FACE('',(#1552),#1119,.F.) ;
#14641=ADVANCED_FACE('',(#1553,#625),#832,.F.) ;
#14642=ADVANCED_FACE('',(#1554),#1120,.F.) ;
#14643=ADVANCED_FACE('',(#1555),#1121,.F.) ;
#14644=ADVANCED_FACE('',(#1556,#626),#833,.F.) ;
#14645=ADVANCED_FACE('',(#1557),#1122,.F.) ;
#14646=ADVANCED_FACE('',(#1558),#1123,.F.) ;
#14647=ADVANCED_FACE('',(#1559,#627),#834,.F.) ;
#14648=ADVANCED_FACE('',(#1560),#1124,.F.) ;
#14649=ADVANCED_FACE('',(#1561),#1125,.F.) ;
#14650=ADVANCED_FACE('',(#1562,#628),#835,.F.) ;
#14651=ADVANCED_FACE('',(#1563),#1126,.F.) ;
#14652=ADVANCED_FACE('',(#1564),#1127,.F.) ;
#14653=ADVANCED_FACE('',(#1565),#14500,.F.) ;
#14654=ADVANCED_FACE('',(#1566),#1128,.F.) ;
#14655=ADVANCED_FACE('',(#1567),#14501,.F.) ;
#14656=ADVANCED_FACE('',(#1568),#1129,.F.) ;
#14657=ADVANCED_FACE('',(#1569),#14502,.F.) ;
#14658=ADVANCED_FACE('',(#1570),#1130,.F.) ;
#14659=ADVANCED_FACE('',(#1571),#14503,.F.) ;
#14660=ADVANCED_FACE('',(#1572),#1131,.F.) ;
#14661=ADVANCED_FACE('',(#1573),#14504,.F.) ;
#14662=ADVANCED_FACE('',(#1574),#1132,.F.) ;
#14663=ADVANCED_FACE('',(#1575),#14505,.F.) ;
#14664=ADVANCED_FACE('',(#1576),#1133,.F.) ;
#14665=ADVANCED_FACE('',(#1577),#14506,.F.) ;
#14666=ADVANCED_FACE('',(#1578),#1134,.F.) ;
#14667=ADVANCED_FACE('',(#1579),#14507,.F.) ;
#14668=ADVANCED_FACE('',(#1580),#1135,.F.) ;
#14669=ADVANCED_FACE('',(#1581),#1136,.F.) ;
#14670=ADVANCED_FACE('',(#1582,#629,#630),#836,.T.) ;
#14671=ADVANCED_FACE('',(#1583),#837,.T.) ;
#14672=ADVANCED_FACE('',(#1584,#631,#632),#838,.T.) ;
#14673=ADVANCED_FACE('',(#1585),#839,.T.) ;
#14674=ADVANCED_FACE('',(#1586,#633,#634,#635,#636,#637),#840,.T.) ;
#14675=ADVANCED_FACE('',(#1587,#638,#639,#640,#641,#642,#643,#644,#645,
#646,#647,#648,#649,#650),#841,.F.) ;
#15494=CLOSED_SHELL('',(#14633,#14634,#14635,#14636,#14637,#14638,#14639,
#14640,#14641,#14642,#14643,#14644,#14645,#14646,#14647,#14648,#14649,#14650,
#14651,#14652,#14653,#14654,#14655,#14656,#14657,#14658,#14659,#14660,#14661,
#14662,#14663,#14664,#14665,#14666,#14667,#14668,#14669,#14670,#14671,#14672,
#14673,#14674,#14675)) ;
#15676=AXIS2_PLACEMENT_3D('',#23013,#17904,#17905) ;
#15677=AXIS2_PLACEMENT_3D('',#23014,#17906,#17907) ;
#15678=AXIS2_PLACEMENT_3D('',#23018,#17909,#17910) ;
#15679=AXIS2_PLACEMENT_3D('',#23019,#17911,#17912) ;
#15680=AXIS2_PLACEMENT_3D('',#23021,#17913,#17914) ;
#15681=AXIS2_PLACEMENT_3D('',#23023,#17916,#17917) ;
#15682=AXIS2_PLACEMENT_3D('',#23027,#17919,#17920) ;
#15683=AXIS2_PLACEMENT_3D('',#23028,#17921,#17922) ;
#15684=AXIS2_PLACEMENT_3D('',#23030,#17923,#17924) ;
#15685=AXIS2_PLACEMENT_3D('',#23032,#17926,#17927) ;
#15686=AXIS2_PLACEMENT_3D('',#23036,#17929,#17930) ;
#15687=AXIS2_PLACEMENT_3D('',#23037,#17931,#17932) ;
#15688=AXIS2_PLACEMENT_3D('',#23039,#17933,#17934) ;
#15689=AXIS2_PLACEMENT_3D('',#23041,#17936,#17937) ;
#15690=AXIS2_PLACEMENT_3D('',#23045,#17939,#17940) ;
#15691=AXIS2_PLACEMENT_3D('',#23046,#17941,#17942) ;
#15692=AXIS2_PLACEMENT_3D('',#23048,#17943,#17944) ;
#15693=AXIS2_PLACEMENT_3D('',#23050,#17946,#17947) ;
#15694=AXIS2_PLACEMENT_3D('',#23052,#17948,#17949) ;
#15695=AXIS2_PLACEMENT_3D('',#23054,#17950,#17951) ;
#15696=AXIS2_PLACEMENT_3D('',#23055,#17952,#17953) ;
#15697=AXIS2_PLACEMENT_3D('',#23057,#17954,#17955) ;
#15698=AXIS2_PLACEMENT_3D('',#23059,#17957,#17958) ;
#15699=AXIS2_PLACEMENT_3D('',#23062,#17960,#17961) ;
#15700=AXIS2_PLACEMENT_3D('',#23063,#17962,#17963) ;
#15701=AXIS2_PLACEMENT_3D('',#23065,#17964,#17965) ;
#15702=AXIS2_PLACEMENT_3D('',#23067,#17966,#17967) ;
#15703=AXIS2_PLACEMENT_3D('',#23068,#17968,#17969) ;
#15704=AXIS2_PLACEMENT_3D('',#23070,#17970,#17971) ;
#15705=AXIS2_PLACEMENT_3D('',#23072,#17973,#17974) ;
#15706=AXIS2_PLACEMENT_3D('',#23075,#17976,#17977) ;
#15707=AXIS2_PLACEMENT_3D('',#23076,#17978,#17979) ;
#15708=AXIS2_PLACEMENT_3D('',#23078,#17980,#17981) ;
#15709=AXIS2_PLACEMENT_3D('',#23080,#17982,#17983) ;
#15710=AXIS2_PLACEMENT_3D('',#23081,#17984,#17985) ;
#15711=AXIS2_PLACEMENT_3D('',#23083,#17986,#17987) ;
#15712=AXIS2_PLACEMENT_3D('',#23085,#17989,#17990) ;
#15713=AXIS2_PLACEMENT_3D('',#23088,#17992,#17993) ;
#15714=AXIS2_PLACEMENT_3D('',#23089,#17994,#17995) ;
#15715=AXIS2_PLACEMENT_3D('',#23091,#17996,#17997) ;
#15716=AXIS2_PLACEMENT_3D('',#23093,#17998,#17999) ;
#15717=AXIS2_PLACEMENT_3D('',#23094,#18000,#18001) ;
#15718=AXIS2_PLACEMENT_3D('',#23096,#18002,#18003) ;
#15719=AXIS2_PLACEMENT_3D('',#23098,#18005,#18006) ;
#15720=AXIS2_PLACEMENT_3D('',#23101,#18008,#18009) ;
#15721=AXIS2_PLACEMENT_3D('',#23102,#18010,#18011) ;
#15722=AXIS2_PLACEMENT_3D('',#23106,#18013,#18014) ;
#15723=AXIS2_PLACEMENT_3D('',#23107,#18015,#18016) ;
#15724=AXIS2_PLACEMENT_3D('',#23109,#18017,#18018) ;
#15725=AXIS2_PLACEMENT_3D('',#23111,#18020,#18021) ;
#15726=AXIS2_PLACEMENT_3D('',#23115,#18023,#18024) ;
#15727=AXIS2_PLACEMENT_3D('',#23116,#18025,#18026) ;
#15728=AXIS2_PLACEMENT_3D('',#23118,#18027,#18028) ;
#15729=AXIS2_PLACEMENT_3D('',#23120,#18030,#18031) ;
#15730=AXIS2_PLACEMENT_3D('',#23124,#18033,#18034) ;
#15731=AXIS2_PLACEMENT_3D('',#23125,#18035,#18036) ;
#15732=AXIS2_PLACEMENT_3D('',#23127,#18037,#18038) ;
#15733=AXIS2_PLACEMENT_3D('',#23129,#18040,#18041) ;
#15734=AXIS2_PLACEMENT_3D('',#23133,#18043,#18044) ;
#15735=AXIS2_PLACEMENT_3D('',#23134,#18045,#18046) ;
#15736=AXIS2_PLACEMENT_3D('',#23136,#18047,#18048) ;
#15737=AXIS2_PLACEMENT_3D('',#23138,#18050,#18051) ;
#15738=AXIS2_PLACEMENT_3D('',#23142,#18053,#18054) ;
#15739=AXIS2_PLACEMENT_3D('',#23143,#18055,#18056) ;
#15740=AXIS2_PLACEMENT_3D('',#23145,#18057,#18058) ;
#15741=AXIS2_PLACEMENT_3D('',#23147,#18060,#18061) ;
#15742=AXIS2_PLACEMENT_3D('',#23151,#18063,#18064) ;
#15743=AXIS2_PLACEMENT_3D('',#23152,#18065,#18066) ;
#15744=AXIS2_PLACEMENT_3D('',#23154,#18067,#18068) ;
#15745=AXIS2_PLACEMENT_3D('',#23156,#18070,#18071) ;
#15746=AXIS2_PLACEMENT_3D('',#23160,#18073,#18074) ;
#15747=AXIS2_PLACEMENT_3D('',#23161,#18075,#18076) ;
#15748=AXIS2_PLACEMENT_3D('',#23163,#18077,#18078) ;
#15749=AXIS2_PLACEMENT_3D('',#23165,#18080,#18081) ;
#15750=AXIS2_PLACEMENT_3D('',#23169,#18083,#18084) ;
#15751=AXIS2_PLACEMENT_3D('',#23170,#18085,#18086) ;
#15752=AXIS2_PLACEMENT_3D('',#23172,#18087,#18088) ;
#15753=AXIS2_PLACEMENT_3D('',#23174,#18090,#18091) ;
#15754=AXIS2_PLACEMENT_3D('',#23176,#18092,#18093) ;
#15755=AXIS2_PLACEMENT_3D('',#23179,#18095,#18096) ;
#15756=AXIS2_PLACEMENT_3D('',#23180,#18097,#18098) ;
#15757=AXIS2_PLACEMENT_3D('',#23189,#18103,#18104) ;
#15758=AXIS2_PLACEMENT_3D('',#23195,#18108,#18109) ;
#15759=AXIS2_PLACEMENT_3D('',#23201,#18113,#18114) ;
#15760=AXIS2_PLACEMENT_3D('',#23204,#18117,#18118) ;
#15761=AXIS2_PLACEMENT_3D('',#23205,#18119,#18120) ;
#17904=DIRECTION('axis',(0.,0.,1.)) ;
#17905=DIRECTION('refdir',(1.,0.,0.)) ;
#17906=DIRECTION('center_axis',(-9.473903143468E-16,1.,0.)) ;
#17907=DIRECTION('ref_axis',(0.,0.,1.)) ;
#17908=DIRECTION('',(-5.92914802803472E-16,0.515038074910058,-0.85716730070211)) ;
#17909=DIRECTION('center_axis',(9.473903143468E-16,-1.,0.)) ;
#17910=DIRECTION('ref_axis',(0.,0.,1.)) ;
#17911=DIRECTION('center_axis',(9.473903143468E-16,-1.,0.)) ;
#17912=DIRECTION('ref_axis',(0.,0.,1.)) ;
#17913=DIRECTION('center_axis',(9.47390314346801E-16,-1.,0.)) ;
#17914=DIRECTION('ref_axis',(0.,0.,1.)) ;
#17915=DIRECTION('',(9.473903143468E-16,-1.,0.)) ;
#17916=DIRECTION('center_axis',(-9.473903143468E-16,1.,0.)) ;
#17917=DIRECTION('ref_axis',(0.,0.,1.)) ;
#17918=DIRECTION('',(-5.92914802803472E-16,0.515038074910058,-0.85716730070211)) ;
#17919=DIRECTION('center_axis',(9.473903143468E-16,-1.,0.)) ;
#17920=DIRECTION('ref_axis',(0.,0.,1.)) ;
#17921=DIRECTION('center_axis',(9.473903143468E-16,-1.,0.)) ;
#17922=DIRECTION('ref_axis',(0.,0.,1.)) ;
#17923=DIRECTION('center_axis',(9.47390314346801E-16,-1.,0.)) ;
#17924=DIRECTION('ref_axis',(0.,0.,1.)) ;
#17925=DIRECTION('',(9.473903143468E-16,-1.,0.)) ;
#17926=DIRECTION('center_axis',(-3.5527136788005E-16,-1.,0.)) ;
#17927=DIRECTION('ref_axis',(0.,0.,-1.)) ;
#17928=DIRECTION('',(-2.87951000497466E-16,-0.515038074910058,0.85716730070211)) ;
#17929=DIRECTION('center_axis',(3.5527136788005E-16,1.,0.)) ;
#17930=DIRECTION('ref_axis',(0.,0.,-1.)) ;
#17931=DIRECTION('center_axis',(3.5527136788005E-16,1.,0.)) ;
#17932=DIRECTION('ref_axis',(0.,0.,-1.)) ;
#17933=DIRECTION('center_axis',(4.2632564145606E-15,1.,0.)) ;
#17934=DIRECTION('ref_axis',(0.,0.,-1.)) ;
#17935=DIRECTION('',(3.5527136788005E-16,1.,0.)) ;
#17936=DIRECTION('center_axis',(-3.5527136788005E-16,-1.,0.)) ;
#17937=DIRECTION('ref_axis',(0.,0.,-1.)) ;
#17938=DIRECTION('',(-2.87951000497466E-16,-0.515038074910058,0.85716730070211)) ;
#17939=DIRECTION('center_axis',(3.5527136788005E-16,1.,0.)) ;
#17940=DIRECTION('ref_axis',(0.,0.,-1.)) ;
#17941=DIRECTION('center_axis',(3.5527136788005E-16,1.,0.)) ;
#17942=DIRECTION('ref_axis',(0.,0.,-1.)) ;
#17943=DIRECTION('center_axis',(4.2632564145606E-15,1.,0.)) ;
#17944=DIRECTION('ref_axis',(0.,0.,-1.)) ;
#17945=DIRECTION('',(3.5527136788005E-16,1.,0.)) ;
#17946=DIRECTION('center_axis',(0.,0.,-1.)) ;
#17947=DIRECTION('ref_axis',(1.,0.,0.)) ;
#17948=DIRECTION('center_axis',(0.,0.,-1.)) ;
#17949=DIRECTION('ref_axis',(1.,0.,0.)) ;
#17950=DIRECTION('center_axis',(0.,0.,-1.)) ;
#17951=DIRECTION('ref_axis',(1.,0.,0.)) ;
#17952=DIRECTION('center_axis',(0.,0.,-1.)) ;
#17953=DIRECTION('ref_axis',(1.,0.,0.)) ;
#17954=DIRECTION('center_axis',(0.,0.,-1.)) ;
#17955=DIRECTION('ref_axis',(1.,0.,0.)) ;
#17956=DIRECTION('',(0.,0.,-1.)) ;
#17957=DIRECTION('center_axis',(0.,0.,-1.)) ;
#17958=DIRECTION('ref_axis',(1.,0.,0.)) ;
#17959=DIRECTION('',(0.,0.,-1.)) ;
#17960=DIRECTION('center_axis',(0.,0.,1.)) ;
#17961=DIRECTION('ref_axis',(1.,0.,0.)) ;
#17962=DIRECTION('center_axis',(0.,0.,-1.)) ;
#17963=DIRECTION('ref_axis',(1.,0.,0.)) ;
#17964=DIRECTION('center_axis',(0.,0.,-1.)) ;
#17965=DIRECTION('ref_axis',(1.,0.,0.)) ;
#17966=DIRECTION('center_axis',(0.,0.,-1.)) ;
#17967=DIRECTION('ref_axis',(1.,0.,0.)) ;
#17968=DIRECTION('center_axis',(0.,0.,-1.)) ;
#17969=DIRECTION('ref_axis',(1.,0.,0.)) ;
#17970=DIRECTION('center_axis',(0.,0.,-1.)) ;
#17971=DIRECTION('ref_axis',(1.,0.,0.)) ;
#17972=DIRECTION('',(0.,0.,-1.)) ;
#17973=DIRECTION('center_axis',(0.,0.,-1.)) ;
#17974=DIRECTION('ref_axis',(1.,0.,0.)) ;
#17975=DIRECTION('',(0.,0.,-1.)) ;
#17976=DIRECTION('center_axis',(0.,0.,1.)) ;
#17977=DIRECTION('ref_axis',(1.,0.,0.)) ;
#17978=DIRECTION('center_axis',(0.,0.,-1.)) ;
#17979=DIRECTION('ref_axis',(1.,0.,0.)) ;
#17980=DIRECTION('center_axis',(0.,0.,-1.)) ;
#17981=DIRECTION('ref_axis',(1.,0.,0.)) ;
#17982=DIRECTION('center_axis',(0.,0.,-1.)) ;
#17983=DIRECTION('ref_axis',(1.,0.,0.)) ;
#17984=DIRECTION('center_axis',(0.,0.,-1.)) ;
#17985=DIRECTION('ref_axis',(1.,0.,0.)) ;
#17986=DIRECTION('center_axis',(0.,0.,-1.)) ;
#17987=DIRECTION('ref_axis',(1.,0.,0.)) ;
#17988=DIRECTION('',(0.,0.,-1.)) ;
#17989=DIRECTION('center_axis',(0.,0.,-1.)) ;
#17990=DIRECTION('ref_axis',(1.,0.,0.)) ;
#17991=DIRECTION('',(0.,0.,-1.)) ;
#17992=DIRECTION('center_axis',(0.,0.,1.)) ;
#17993=DIRECTION('ref_axis',(1.,0.,0.)) ;
#17994=DIRECTION('center_axis',(0.,0.,-1.)) ;
#17995=DIRECTION('ref_axis',(1.,0.,0.)) ;
#17996=DIRECTION('center_axis',(0.,0.,-1.)) ;
#17997=DIRECTION('ref_axis',(1.,0.,0.)) ;
#17998=DIRECTION('center_axis',(0.,0.,-1.)) ;
#17999=DIRECTION('ref_axis',(1.,0.,0.)) ;
#18000=DIRECTION('center_axis',(0.,0.,-1.)) ;
#18001=DIRECTION('ref_axis',(1.,0.,0.)) ;
#18002=DIRECTION('center_axis',(0.,0.,-1.)) ;
#18003=DIRECTION('ref_axis',(1.,0.,0.)) ;
#18004=DIRECTION('',(0.,0.,-1.)) ;
#18005=DIRECTION('center_axis',(0.,0.,-1.)) ;
#18006=DIRECTION('ref_axis',(1.,0.,0.)) ;
#18007=DIRECTION('',(0.,0.,-1.)) ;
#18008=DIRECTION('center_axis',(0.,0.,1.)) ;
#18009=DIRECTION('ref_axis',(1.,0.,0.)) ;
#18010=DIRECTION('center_axis',(0.,0.,-1.)) ;
#18011=DIRECTION('ref_axis',(-1.,0.,0.)) ;
#18012=DIRECTION('',(0.85716730070211,-1.04972719113862E-16,-0.515038074910058)) ;
#18013=DIRECTION('center_axis',(0.,0.,1.)) ;
#18014=DIRECTION('ref_axis',(-1.,0.,0.)) ;
#18015=DIRECTION('center_axis',(0.,0.,1.)) ;
#18016=DIRECTION('ref_axis',(-1.,0.,0.)) ;
#18017=DIRECTION('center_axis',(0.,0.,1.)) ;
#18018=DIRECTION('ref_axis',(-1.,0.,0.)) ;
#18019=DIRECTION('',(0.,0.,1.)) ;
#18020=DIRECTION('center_axis',(0.,0.,-1.)) ;
#18021=DIRECTION('ref_axis',(-1.,0.,0.)) ;
#18022=DIRECTION('',(0.85716730070211,-1.04972719113862E-16,-0.515038074910058)) ;
#18023=DIRECTION('center_axis',(0.,0.,1.)) ;
#18024=DIRECTION('ref_axis',(-1.,0.,0.)) ;
#18025=DIRECTION('center_axis',(0.,0.,1.)) ;
#18026=DIRECTION('ref_axis',(-1.,0.,0.)) ;
#18027=DIRECTION('center_axis',(0.,0.,-1.)) ;
#18028=DIRECTION('ref_axis',(-1.,0.,0.)) ;
#18029=DIRECTION('',(0.,0.,1.)) ;
#18030=DIRECTION('center_axis',(0.,0.,-1.)) ;
#18031=DIRECTION('ref_axis',(-1.,0.,0.)) ;
#18032=DIRECTION('',(0.85716730070211,-1.04972719113862E-16,-0.515038074910058)) ;
#18033=DIRECTION('center_axis',(0.,0.,1.)) ;
#18034=DIRECTION('ref_axis',(-1.,0.,0.)) ;
#18035=DIRECTION('center_axis',(0.,0.,1.)) ;
#18036=DIRECTION('ref_axis',(-1.,0.,0.)) ;
#18037=DIRECTION('center_axis',(0.,0.,-1.)) ;
#18038=DIRECTION('ref_axis',(-1.,0.,0.)) ;
#18039=DIRECTION('',(0.,0.,1.)) ;
#18040=DIRECTION('center_axis',(0.,0.,-1.)) ;
#18041=DIRECTION('ref_axis',(-1.,0.,0.)) ;
#18042=DIRECTION('',(0.85716730070211,-1.04972719113862E-16,-0.515038074910058)) ;
#18043=DIRECTION('center_axis',(0.,0.,1.)) ;
#18044=DIRECTION('ref_axis',(-1.,0.,0.)) ;
#18045=DIRECTION('center_axis',(0.,0.,1.)) ;
#18046=DIRECTION('ref_axis',(-1.,0.,0.)) ;
#18047=DIRECTION('center_axis',(0.,0.,-1.)) ;
#18048=DIRECTION('ref_axis',(-1.,0.,0.)) ;
#18049=DIRECTION('',(0.,0.,1.)) ;
#18050=DIRECTION('center_axis',(0.,0.,-1.)) ;
#18051=DIRECTION('ref_axis',(-1.,0.,0.)) ;
#18052=DIRECTION('',(0.85716730070211,-1.04972719113862E-16,-0.515038074910058)) ;
#18053=DIRECTION('center_axis',(0.,0.,1.)) ;
#18054=DIRECTION('ref_axis',(-1.,0.,0.)) ;
#18055=DIRECTION('center_axis',(0.,0.,1.)) ;
#18056=DIRECTION('ref_axis',(-1.,0.,0.)) ;
#18057=DIRECTION('center_axis',(0.,0.,-1.)) ;
#18058=DIRECTION('ref_axis',(-1.,0.,0.)) ;
#18059=DIRECTION('',(0.,0.,1.)) ;
#18060=DIRECTION('center_axis',(0.,0.,-1.)) ;
#18061=DIRECTION('ref_axis',(-1.,0.,0.)) ;
#18062=DIRECTION('',(0.85716730070211,-1.04972719113862E-16,-0.515038074910058)) ;
#18063=DIRECTION('center_axis',(0.,0.,1.)) ;
#18064=DIRECTION('ref_axis',(-1.,0.,0.)) ;
#18065=DIRECTION('center_axis',(0.,0.,1.)) ;
#18066=DIRECTION('ref_axis',(-1.,0.,0.)) ;
#18067=DIRECTION('center_axis',(0.,0.,-1.)) ;
#18068=DIRECTION('ref_axis',(-1.,0.,0.)) ;
#18069=DIRECTION('',(0.,0.,1.)) ;
#18070=DIRECTION('center_axis',(0.,0.,-1.)) ;
#18071=DIRECTION('ref_axis',(-1.,0.,0.)) ;
#18072=DIRECTION('',(0.85716730070211,-1.04972719113862E-16,-0.515038074910058)) ;
#18073=DIRECTION('center_axis',(0.,0.,1.)) ;
#18074=DIRECTION('ref_axis',(-1.,0.,0.)) ;
#18075=DIRECTION('center_axis',(0.,0.,1.)) ;
#18076=DIRECTION('ref_axis',(-1.,0.,0.)) ;
#18077=DIRECTION('center_axis',(0.,0.,-1.)) ;
#18078=DIRECTION('ref_axis',(-1.,0.,0.)) ;
#18079=DIRECTION('',(0.,0.,1.)) ;
#18080=DIRECTION('center_axis',(0.,0.,-1.)) ;
#18081=DIRECTION('ref_axis',(-1.,0.,0.)) ;
#18082=DIRECTION('',(0.85716730070211,-1.04972719113862E-16,-0.515038074910058)) ;
#18083=DIRECTION('center_axis',(0.,0.,1.)) ;
#18084=DIRECTION('ref_axis',(-1.,0.,0.)) ;
#18085=DIRECTION('center_axis',(0.,0.,1.)) ;
#18086=DIRECTION('ref_axis',(-1.,0.,0.)) ;
#18087=DIRECTION('center_axis',(0.,0.,1.)) ;
#18088=DIRECTION('ref_axis',(-1.,0.,0.)) ;
#18089=DIRECTION('',(0.,0.,1.)) ;
#18090=DIRECTION('center_axis',(0.,0.,-1.)) ;
#18091=DIRECTION('ref_axis',(1.,0.,0.)) ;
#18092=DIRECTION('center_axis',(0.,0.,-1.)) ;
#18093=DIRECTION('ref_axis',(1.,0.,0.)) ;
#18094=DIRECTION('',(0.,0.,-1.)) ;
#18095=DIRECTION('center_axis',(0.,0.,1.)) ;
#18096=DIRECTION('ref_axis',(1.,0.,0.)) ;
#18097=DIRECTION('center_axis',(-4.2632564145606E-15,-1.,0.)) ;
#18098=DIRECTION('ref_axis',(-1.,4.2632564145606E-15,0.)) ;
#18099=DIRECTION('',(1.,-4.2632564145606E-15,0.)) ;
#18100=DIRECTION('',(0.,0.,-1.)) ;
#18101=DIRECTION('',(-1.,4.2632564145606E-15,0.)) ;
#18102=DIRECTION('',(0.,0.,-1.)) ;
#18103=DIRECTION('center_axis',(1.,-2.66453525910036E-16,0.)) ;
#18104=DIRECTION('ref_axis',(-2.66453525910036E-16,-1.,0.)) ;
#18105=DIRECTION('',(2.66453525910036E-16,1.,0.)) ;
#18106=DIRECTION('',(-2.66453525910036E-16,-1.,0.)) ;
#18107=DIRECTION('',(0.,0.,-1.)) ;
#18108=DIRECTION('center_axis',(-9.47390314346801E-16,1.,0.)) ;
#18109=DIRECTION('ref_axis',(1.,9.47390314346801E-16,0.)) ;
#18110=DIRECTION('',(1.,9.47390314346801E-16,0.)) ;
#18111=DIRECTION('',(1.,9.47390314346801E-16,0.)) ;
#18112=DIRECTION('',(0.,0.,-1.)) ;
#18113=DIRECTION('center_axis',(-1.,1.68753899743024E-15,0.)) ;
#18114=DIRECTION('ref_axis',(1.68753899743024E-15,1.,0.)) ;
#18115=DIRECTION('',(-1.68753899743024E-15,-1.,0.)) ;
#18116=DIRECTION('',(1.68753899743024E-15,1.,0.)) ;
#18117=DIRECTION('center_axis',(0.,0.,1.)) ;
#18118=DIRECTION('ref_axis',(1.,0.,0.)) ;
#18119=DIRECTION('center_axis',(0.,0.,1.)) ;
#18120=DIRECTION('ref_axis',(1.,0.,0.)) ;
#23013=CARTESIAN_POINT('',(0.,0.,0.)) ;
#23014=CARTESIAN_POINT('Origin',(-45.0000000000005,385.343736383858,-12.)) ;
#23015=CARTESIAN_POINT('',(-45.0000000000005,383.888531181086,-12.)) ;
#23016=CARTESIAN_POINT('',(-45.0000000000005,386.45,-16.263)) ;
#23017=CARTESIAN_POINT('',(-45.0000000000005,385.343736383858,-14.4218681615831)) ;
#23018=CARTESIAN_POINT('Origin',(-45.0000000000005,386.45,-12.)) ;
#23019=CARTESIAN_POINT('Origin',(-45.0000000000005,405.45,-12.)) ;
#23020=CARTESIAN_POINT('',(-45.0000000000005,409.45,-16.263)) ;
#23021=CARTESIAN_POINT('Origin',(-45.0000000000005,409.45,-12.)) ;
#23022=CARTESIAN_POINT('',(-45.0000000000005,405.45,-16.263)) ;
#23023=CARTESIAN_POINT('Origin',(44.9999999999989,385.343736383858,-12.)) ;
#23024=CARTESIAN_POINT('',(44.9999999999989,383.888531181086,-12.)) ;
#23025=CARTESIAN_POINT('',(44.9999999999989,386.45,-16.263)) ;
#23026=CARTESIAN_POINT('',(44.9999999999989,385.343736383858,-14.4218681615831)) ;
#23027=CARTESIAN_POINT('Origin',(44.9999999999989,386.45,-12.)) ;
#23028=CARTESIAN_POINT('Origin',(44.9999999999989,405.45,-12.)) ;
#23029=CARTESIAN_POINT('',(44.9999999999989,409.45,-16.263)) ;
#23030=CARTESIAN_POINT('Origin',(44.9999999999989,409.45,-12.)) ;
#23031=CARTESIAN_POINT('',(44.9999999999989,405.45,-16.263)) ;
#23032=CARTESIAN_POINT('Origin',(-44.9999999999999,228.556263616143,-12.)) ;
#23033=CARTESIAN_POINT('',(-44.9999999999999,230.011468818915,-12.)) ;
#23034=CARTESIAN_POINT('',(-44.9999999999999,227.45,-7.737)) ;
#23035=CARTESIAN_POINT('',(-44.9999999999999,228.556263616143,-9.57813183841693)) ;
#23036=CARTESIAN_POINT('Origin',(-44.9999999999999,227.45,-12.)) ;
#23037=CARTESIAN_POINT('Origin',(-44.9999999999999,208.45,-12.)) ;
#23038=CARTESIAN_POINT('',(-44.9999999999999,209.449999999999,-7.737)) ;
#23039=CARTESIAN_POINT('Origin',(-44.9999999999999,209.449999999999,-12.)) ;
#23040=CARTESIAN_POINT('',(-44.9999999999999,208.45,-7.737)) ;
#23041=CARTESIAN_POINT('Origin',(44.9999999999995,228.556263616143,-12.)) ;
#23042=CARTESIAN_POINT('',(44.9999999999995,230.011468818915,-12.)) ;
#23043=CARTESIAN_POINT('',(44.9999999999995,227.45,-7.737)) ;
#23044=CARTESIAN_POINT('',(44.9999999999995,228.556263616143,-9.57813183841693)) ;
#23045=CARTESIAN_POINT('Origin',(44.9999999999995,227.45,-12.)) ;
#23046=CARTESIAN_POINT('Origin',(44.9999999999995,208.45,-12.)) ;
#23047=CARTESIAN_POINT('',(44.9999999999995,209.449999999999,-7.737)) ;
#23048=CARTESIAN_POINT('Origin',(44.9999999999995,209.449999999999,-12.)) ;
#23049=CARTESIAN_POINT('',(44.9999999999995,208.45,-7.737)) ;
#23050=CARTESIAN_POINT('Origin',(-62.9999999999999,239.45,-10.)) ;
#23051=CARTESIAN_POINT('',(-71.9999999999999,239.45,-10.)) ;
#23052=CARTESIAN_POINT('Origin',(-62.9999999999999,239.45,-10.)) ;
#23053=CARTESIAN_POINT('',(-68.4999999999999,239.45,-10.)) ;
#23054=CARTESIAN_POINT('Origin',(-62.9999999999999,239.45,-10.)) ;
#23055=CARTESIAN_POINT('Origin',(-62.9999999999999,239.45,-5.)) ;
#23056=CARTESIAN_POINT('',(-71.9999999999999,239.45,0.)) ;
#23057=CARTESIAN_POINT('Origin',(-62.9999999999999,239.45,0.)) ;
#23058=CARTESIAN_POINT('',(-71.9999999999999,239.45,-5.)) ;
#23059=CARTESIAN_POINT('Origin',(-62.9999999999999,239.45,-19.)) ;
#23060=CARTESIAN_POINT('',(-68.4999999999999,239.45,-24.)) ;
#23061=CARTESIAN_POINT('',(-68.4999999999999,239.45,-19.)) ;
#23062=CARTESIAN_POINT('Origin',(-62.9999999999999,239.45,-24.)) ;
#23063=CARTESIAN_POINT('Origin',(63.,379.45,-10.)) ;
#23064=CARTESIAN_POINT('',(54.,379.45,-10.)) ;
#23065=CARTESIAN_POINT('Origin',(63.,379.45,-10.)) ;
#23066=CARTESIAN_POINT('',(57.5,379.45,-10.)) ;
#23067=CARTESIAN_POINT('Origin',(63.,379.45,-10.)) ;
#23068=CARTESIAN_POINT('Origin',(63.,379.45,-5.)) ;
#23069=CARTESIAN_POINT('',(54.,379.45,0.)) ;
#23070=CARTESIAN_POINT('Origin',(63.,379.45,0.)) ;
#23071=CARTESIAN_POINT('',(54.,379.45,-5.)) ;
#23072=CARTESIAN_POINT('Origin',(63.,379.45,-19.)) ;
#23073=CARTESIAN_POINT('',(57.5,379.45,-24.)) ;
#23074=CARTESIAN_POINT('',(57.5,379.45,-19.)) ;
#23075=CARTESIAN_POINT('Origin',(63.,379.45,-24.)) ;
#23076=CARTESIAN_POINT('Origin',(63.,239.45,-10.)) ;
#23077=CARTESIAN_POINT('',(54.,239.45,-10.)) ;
#23078=CARTESIAN_POINT('Origin',(63.,239.45,-10.)) ;
#23079=CARTESIAN_POINT('',(57.5,239.45,-10.)) ;
#23080=CARTESIAN_POINT('Origin',(63.,239.45,-10.)) ;
#23081=CARTESIAN_POINT('Origin',(63.,239.45,-5.)) ;
#23082=CARTESIAN_POINT('',(54.,239.45,0.)) ;
#23083=CARTESIAN_POINT('Origin',(63.,239.45,0.)) ;
#23084=CARTESIAN_POINT('',(54.,239.45,-5.)) ;
#23085=CARTESIAN_POINT('Origin',(63.,239.45,-19.)) ;
#23086=CARTESIAN_POINT('',(57.5,239.45,-24.)) ;
#23087=CARTESIAN_POINT('',(57.5,239.45,-19.)) ;
#23088=CARTESIAN_POINT('Origin',(63.,239.45,-24.)) ;
#23089=CARTESIAN_POINT('Origin',(-62.9999999999999,379.45,-10.)) ;
#23090=CARTESIAN_POINT('',(-71.9999999999999,379.45,-10.)) ;
#23091=CARTESIAN_POINT('Origin',(-62.9999999999999,379.45,-10.)) ;
#23092=CARTESIAN_POINT('',(-68.4999999999999,379.45,-10.)) ;
#23093=CARTESIAN_POINT('Origin',(-62.9999999999999,379.45,-10.)) ;
#23094=CARTESIAN_POINT('Origin',(-62.9999999999999,379.45,-5.)) ;
#23095=CARTESIAN_POINT('',(-71.9999999999999,379.45,0.)) ;
#23096=CARTESIAN_POINT('Origin',(-62.9999999999999,379.45,0.)) ;
#23097=CARTESIAN_POINT('',(-71.9999999999999,379.45,-5.)) ;
#23098=CARTESIAN_POINT('Origin',(-62.9999999999999,379.45,-19.)) ;
#23099=CARTESIAN_POINT('',(-68.4999999999999,379.45,-24.)) ;
#23100=CARTESIAN_POINT('',(-68.4999999999999,379.45,-19.)) ;
#23101=CARTESIAN_POINT('Origin',(-62.9999999999999,379.45,-24.)) ;
#23102=CARTESIAN_POINT('Origin',(45.,354.45,-13.0085799786045)) ;
#23103=CARTESIAN_POINT('',(45.,354.45,-12.0171599572091)) ;
#23104=CARTESIAN_POINT('',(48.3,354.45,-14.)) ;
#23105=CARTESIAN_POINT('',(46.65,354.45,-13.0085799786045)) ;
#23106=CARTESIAN_POINT('Origin',(45.,354.45,-14.)) ;
#23107=CARTESIAN_POINT('Origin',(45.,354.45,-22.)) ;
#23108=CARTESIAN_POINT('',(48.3,354.45,-24.)) ;
#23109=CARTESIAN_POINT('Origin',(45.,354.45,-24.)) ;
#23110=CARTESIAN_POINT('',(48.3,354.45,-22.)) ;
#23111=CARTESIAN_POINT('Origin',(-5.51091059616309E-15,399.45,-13.3540332243106)) ;
#23112=CARTESIAN_POINT('',(-5.67105257905314E-15,399.45,-12.4873333915981)) ;
#23113=CARTESIAN_POINT('',(2.51749999999999,399.45,-14.)) ;
#23114=CARTESIAN_POINT('',(1.44243074893997,399.45,-13.3540332243106)) ;
#23115=CARTESIAN_POINT('Origin',(-5.51091059616309E-15,399.45,-14.)) ;
#23116=CARTESIAN_POINT('Origin',(-5.51091059616309E-15,399.45,-22.)) ;
#23117=CARTESIAN_POINT('',(2.51749999999999,399.45,-24.)) ;
#23118=CARTESIAN_POINT('Origin',(-5.51091059616309E-15,399.45,-24.)) ;
#23119=CARTESIAN_POINT('',(2.51749999999999,399.45,-22.)) ;
#23120=CARTESIAN_POINT('Origin',(-45.,354.45,-13.3540332243106)) ;
#23121=CARTESIAN_POINT('',(-45.,354.45,-12.4873333915981)) ;
#23122=CARTESIAN_POINT('',(-42.4825,354.45,-14.)) ;
#23123=CARTESIAN_POINT('',(-43.55756925106,354.45,-13.3540332243106)) ;
#23124=CARTESIAN_POINT('Origin',(-45.,354.45,-14.)) ;
#23125=CARTESIAN_POINT('Origin',(-45.,354.45,-22.)) ;
#23126=CARTESIAN_POINT('',(-42.4825,354.45,-24.)) ;
#23127=CARTESIAN_POINT('Origin',(-45.,354.45,-24.)) ;
#23128=CARTESIAN_POINT('',(-42.4825,354.45,-22.)) ;
#23129=CARTESIAN_POINT('Origin',(0.,309.45,-13.3540332243106)) ;
#23130=CARTESIAN_POINT('',(-1.60141982890047E-16,309.45,-12.4873333915981)) ;
#23131=CARTESIAN_POINT('',(2.5175,309.45,-14.)) ;
#23132=CARTESIAN_POINT('',(1.44243074893998,309.45,-13.3540332243106)) ;
#23133=CARTESIAN_POINT('Origin',(0.,309.45,-14.)) ;
#23134=CARTESIAN_POINT('Origin',(0.,309.45,-22.)) ;
#23135=CARTESIAN_POINT('',(2.5175,309.45,-24.)) ;
#23136=CARTESIAN_POINT('Origin',(0.,309.45,-24.)) ;
#23137=CARTESIAN_POINT('',(2.5175,309.45,-22.)) ;
#23138=CARTESIAN_POINT('Origin',(-31.8198051533946,322.630194846605,-13.3540332243106)) ;
#23139=CARTESIAN_POINT('',(-31.8198051533946,322.630194846605,-12.4873333915981)) ;
#23140=CARTESIAN_POINT('',(-29.3023051533946,322.630194846605,-14.)) ;
#23141=CARTESIAN_POINT('',(-30.3773744044546,322.630194846605,-13.3540332243106)) ;
#23142=CARTESIAN_POINT('Origin',(-31.8198051533946,322.630194846605,-14.)) ;
#23143=CARTESIAN_POINT('Origin',(-31.8198051533946,322.630194846605,-22.)) ;
#23144=CARTESIAN_POINT('',(-29.3023051533946,322.630194846605,-24.)) ;
#23145=CARTESIAN_POINT('Origin',(-31.8198051533946,322.630194846605,-24.)) ;
#23146=CARTESIAN_POINT('',(-29.3023051533946,322.630194846605,-22.)) ;
#23147=CARTESIAN_POINT('Origin',(-31.8198051533946,386.269805153395,-13.3540332243106)) ;
#23148=CARTESIAN_POINT('',(-31.8198051533946,386.269805153395,-12.4873333915981)) ;
#23149=CARTESIAN_POINT('',(-29.3023051533946,386.269805153395,-14.)) ;
#23150=CARTESIAN_POINT('',(-30.3773744044546,386.269805153395,-13.3540332243106)) ;
#23151=CARTESIAN_POINT('Origin',(-31.8198051533946,386.269805153395,-14.)) ;
#23152=CARTESIAN_POINT('Origin',(-31.8198051533946,386.269805153395,-22.)) ;
#23153=CARTESIAN_POINT('',(-29.3023051533946,386.269805153395,-24.)) ;
#23154=CARTESIAN_POINT('Origin',(-31.8198051533946,386.269805153395,-24.)) ;
#23155=CARTESIAN_POINT('',(-29.3023051533946,386.269805153395,-22.)) ;
#23156=CARTESIAN_POINT('Origin',(31.8198051533946,386.269805153395,-13.3540332243106)) ;
#23157=CARTESIAN_POINT('',(31.8198051533946,386.269805153395,-12.4873333915981)) ;
#23158=CARTESIAN_POINT('',(34.3373051533946,386.269805153395,-14.)) ;
#23159=CARTESIAN_POINT('',(33.2622359023346,386.269805153395,-13.3540332243106)) ;
#23160=CARTESIAN_POINT('Origin',(31.8198051533946,386.269805153395,-14.)) ;
#23161=CARTESIAN_POINT('Origin',(31.8198051533946,386.269805153395,-22.)) ;
#23162=CARTESIAN_POINT('',(34.3373051533946,386.269805153395,-24.)) ;
#23163=CARTESIAN_POINT('Origin',(31.8198051533946,386.269805153395,-24.)) ;
#23164=CARTESIAN_POINT('',(34.3373051533946,386.269805153395,-22.)) ;
#23165=CARTESIAN_POINT('Origin',(31.8198051533946,322.630194846605,-13.0085799786045)) ;
#23166=CARTESIAN_POINT('',(31.8198051533946,322.630194846605,-12.0171599572091)) ;
#23167=CARTESIAN_POINT('',(35.1198051533946,322.630194846605,-14.)) ;
#23168=CARTESIAN_POINT('',(33.4698051533946,322.630194846605,-13.0085799786045)) ;
#23169=CARTESIAN_POINT('Origin',(31.8198051533946,322.630194846605,-14.)) ;
#23170=CARTESIAN_POINT('Origin',(31.8198051533946,322.630194846605,-22.)) ;
#23171=CARTESIAN_POINT('',(35.1198051533946,322.630194846605,-24.)) ;
#23172=CARTESIAN_POINT('Origin',(31.8198051533946,322.630194846605,-24.)) ;
#23173=CARTESIAN_POINT('',(35.1198051533946,322.630194846605,-22.)) ;
#23174=CARTESIAN_POINT('Origin',(0.,354.45,0.)) ;
#23175=CARTESIAN_POINT('',(-37.5,354.45,0.)) ;
#23176=CARTESIAN_POINT('Origin',(0.,354.45,0.)) ;
#23177=CARTESIAN_POINT('',(-37.5,354.45,-24.)) ;
#23178=CARTESIAN_POINT('',(-37.5,354.45,0.)) ;
#23179=CARTESIAN_POINT('Origin',(0.,354.45,-24.)) ;
#23180=CARTESIAN_POINT('Origin',(75.,209.449999999999,0.)) ;
#23181=CARTESIAN_POINT('',(-75.0000000000002,209.45,0.)) ;
#23182=CARTESIAN_POINT('',(75.,209.449999999999,0.)) ;
#23183=CARTESIAN_POINT('',(-100.,209.45,0.)) ;
#23184=CARTESIAN_POINT('',(-75.0000000000002,209.45,-24.)) ;
#23185=CARTESIAN_POINT('',(-75.0000000000002,209.45,0.)) ;
#23186=CARTESIAN_POINT('',(75.,209.449999999999,-24.)) ;
#23187=CARTESIAN_POINT('',(-100.,209.45,-24.)) ;
#23188=CARTESIAN_POINT('',(75.,209.449999999999,0.)) ;
#23189=CARTESIAN_POINT('Origin',(75.0000000000001,409.45,0.)) ;
#23190=CARTESIAN_POINT('',(75.0000000000001,409.45,0.)) ;
#23191=CARTESIAN_POINT('',(75.,209.449999999999,0.)) ;
#23192=CARTESIAN_POINT('',(75.0000000000001,409.45,-24.)) ;
#23193=CARTESIAN_POINT('',(75.,209.449999999999,-24.)) ;
#23194=CARTESIAN_POINT('',(75.0000000000001,409.45,0.)) ;
#23195=CARTESIAN_POINT('Origin',(-74.9999999999999,409.45,0.)) ;
#23196=CARTESIAN_POINT('',(-74.9999999999999,409.45,0.)) ;
#23197=CARTESIAN_POINT('',(-74.9999999999999,409.45,0.)) ;
#23198=CARTESIAN_POINT('',(-74.9999999999999,409.45,-24.)) ;
#23199=CARTESIAN_POINT('',(-74.9999999999999,409.45,-24.)) ;
#23200=CARTESIAN_POINT('',(-74.9999999999999,409.45,0.)) ;
#23201=CARTESIAN_POINT('Origin',(-75.0000000000002,209.45,0.)) ;
#23202=CARTESIAN_POINT('',(-74.9999999999999,409.45,0.)) ;
#23203=CARTESIAN_POINT('',(-74.9999999999999,409.45,-24.)) ;
#23204=CARTESIAN_POINT('Origin',(-6.21724893790088E-14,309.45,0.)) ;
#23205=CARTESIAN_POINT('Origin',(-6.21724893790088E-14,309.45,-24.)) ;
#63792=UNCERTAINTY_MEASURE_WITH_UNIT(LENGTH_MEASURE(0.01),#63825,
'DISTANCE_ACCURACY_VALUE',
'Maximum model space distance between geometric entities at asserted c
onnectivities') ;
#63807=UNCERTAINTY_MEASURE_WITH_UNIT(LENGTH_MEASURE(0.01),#63825,
'DISTANCE_ACCURACY_VALUE',
'Maximum model space distance between geometric entities at asserted c
onnectivities') ;
#63809=(
GEOMETRIC_REPRESENTATION_CONTEXT(3)
GLOBAL_UNCERTAINTY_ASSIGNED_CONTEXT((#63792))
GLOBAL_UNIT_ASSIGNED_CONTEXT((#63825,#63827,#63828))
REPRESENTATION_CONTEXT('','3D')
) ;
#63824=(
GEOMETRIC_REPRESENTATION_CONTEXT(3)
GLOBAL_UNCERTAINTY_ASSIGNED_CONTEXT((#63807))
GLOBAL_UNIT_ASSIGNED_CONTEXT((#63825,#63827,#63828))
REPRESENTATION_CONTEXT('','3D')
) ;
#63825=(
LENGTH_UNIT()
NAMED_UNIT(*)
SI_UNIT(.MILLI.,.METRE.)
) ;
#63827=(
NAMED_UNIT(*)
PLANE_ANGLE_UNIT()
SI_UNIT($,.RADIAN.)
) ;
#63828=(
NAMED_UNIT(*)
SI_UNIT($,.STERADIAN.)
SOLID_ANGLE_UNIT()
) ;
#63830=SHAPE_DEFINITION_REPRESENTATION(#63846,#63879) ;
#63846=PRODUCT_DEFINITION_SHAPE('',$,#63896) ;
#63879=SHAPE_REPRESENTATION('',(#15676),#63809) ;
#63894=PRODUCT_DEFINITION_CONTEXT('part definition',#63944,'design') ;
#63896=PRODUCT_DEFINITION('Back_Plate','Back_Plate',#63912,#63894) ;
#63912=PRODUCT_DEFINITION_FORMATION('',$,#63947) ;
#63944=APPLICATION_CONTEXT(
'Core Data for Automotive Mechanical Design Process') ;
#63945=PRODUCT_CONTEXT('part definition',#63944,'mechanical') ;
#63947=PRODUCT('Back_Plate','Back_Plate',$,(#63945)) ;
#63963=PRESENTATION_STYLE_ASSIGNMENT((#63968)) ;
#63968=SURFACE_STYLE_USAGE(.BOTH.,#63973) ;
#63973=SURFACE_SIDE_STYLE('',(#63978)) ;
#63978=SURFACE_STYLE_FILL_AREA(#63983) ;
#63983=FILL_AREA_STYLE('Opaque(160,160,160)',(#63988)) ;
#63988=FILL_AREA_STYLE_COLOUR('Opaque(160,160,160)',#63993) ;
#63993=COLOUR_RGB('Opaque(160,160,160)', 0.09019608, 0.27058824, 0.51372549) ;
ENDSEC;
END-ISO-10303-21;
